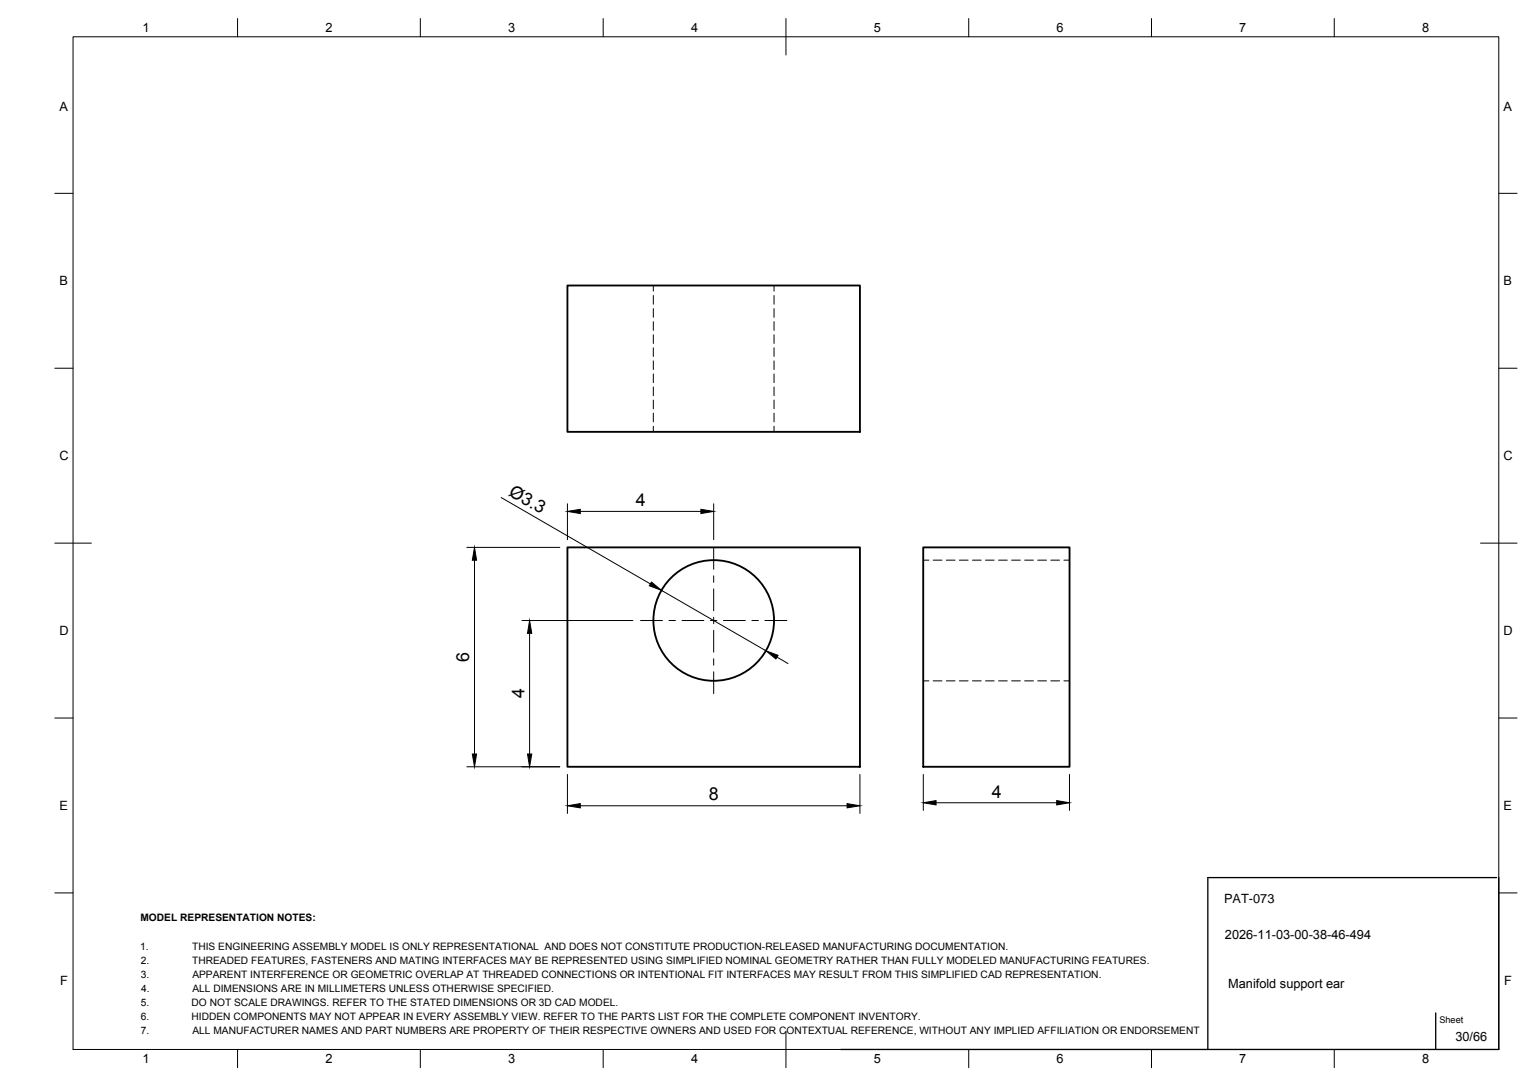
ISO-10303-21;
HEADER;
/* Generated by software containing ST-Developer
 * from STEP Tools, Inc. (www.steptools.com) 
 */

FILE_DESCRIPTION(
/* description */ ('Manual piston pump'),
/* implementation_level */ '2;1');

FILE_NAME(
/* name */ 'Manifold support ear.step',
/* time_stamp */ '2026-11-02T16:54:23-08:00',
/* author */ (''),
/* organization */ (''),
/* preprocessor_version */ 'ST-DEVELOPER v20.2',
/* originating_system */ 'Autodesk Translation Framework v15.17.0.0',
/* authorisation */ '');

FILE_SCHEMA (('AUTOMOTIVE_DESIGN { 1 0 10303 214 3 1 1 }'));
ENDSEC;

DATA;
#10=MECHANICAL_DESIGN_GEOMETRIC_PRESENTATION_REPRESENTATION('',(#732),#19043);
#598=SHAPE_REPRESENTATION_RELATIONSHIP('SRR','None',#19346,#661);
#661=ADVANCED_BREP_SHAPE_REPRESENTATION('',(#802),#19013);
#732=STYLED_ITEM('',(#19661),#802);
#802=MANIFOLD_SOLID_BREP('Body1',#9518);
#993=FACE_BOUND('',#2411,.T.);
#994=FACE_BOUND('',#2413,.T.);
#1230=CYLINDRICAL_SURFACE('',#11012,0.165);
#1664=FACE_OUTER_BOUND('',#2405,.T.);
#1665=FACE_OUTER_BOUND('',#2406,.T.);
#1666=FACE_OUTER_BOUND('',#2407,.T.);
#1667=FACE_OUTER_BOUND('',#2408,.T.);
#1668=FACE_OUTER_BOUND('',#2409,.T.);
#1669=FACE_OUTER_BOUND('',#2410,.T.);
#1670=FACE_OUTER_BOUND('',#2412,.T.);
#2405=EDGE_LOOP('',(#7799,#7800,#7801,#7802));
#2406=EDGE_LOOP('',(#7803,#7804,#7805,#7806));
#2407=EDGE_LOOP('',(#7807,#7808,#7809,#7810));
#2408=EDGE_LOOP('',(#7811,#7812,#7813,#7814));
#2409=EDGE_LOOP('',(#7815,#7816,#7817,#7818));
#2410=EDGE_LOOP('',(#7819,#7820,#7821,#7822));
#2411=EDGE_LOOP('',(#7823));
#2412=EDGE_LOOP('',(#7824,#7825,#7826,#7827));
#2413=EDGE_LOOP('',(#7828));
#3007=CIRCLE('',#11013,0.165);
#3008=CIRCLE('',#11014,0.165);
#3520=LINE('',#17795,#4124);
#3521=LINE('',#17800,#4125);
#3522=LINE('',#17802,#4126);
#3523=LINE('',#17804,#4127);
#3524=LINE('',#17805,#4128);
#3525=LINE('',#17808,#4129);
#3526=LINE('',#17810,#4130);
#3527=LINE('',#17811,#4131);
#3528=LINE('',#17814,#4132);
#3529=LINE('',#17816,#4133);
#3530=LINE('',#17817,#4134);
#3531=LINE('',#17819,#4135);
#3532=LINE('',#17820,#4136);
#4124=VECTOR('',#13410,0.165);
#4125=VECTOR('',#13415,1.);
#4126=VECTOR('',#13416,1.);
#4127=VECTOR('',#13417,1.);
#4128=VECTOR('',#13418,1.);
#4129=VECTOR('',#13421,1.);
#4130=VECTOR('',#13422,1.);
#4131=VECTOR('',#13423,1.);
#4132=VECTOR('',#13426,1.);
#4133=VECTOR('',#13427,1.);
#4134=VECTOR('',#13428,1.);
#4135=VECTOR('',#13431,1.);
#4136=VECTOR('',#13432,1.);
#4870=VERTEX_POINT('',#17792);
#4871=VERTEX_POINT('',#17794);
#4872=VERTEX_POINT('',#17798);
#4873=VERTEX_POINT('',#17799);
#4874=VERTEX_POINT('',#17801);
#4875=VERTEX_POINT('',#17803);
#4876=VERTEX_POINT('',#17807);
#4877=VERTEX_POINT('',#17809);
#4878=VERTEX_POINT('',#17813);
#4879=VERTEX_POINT('',#17815);
#5886=EDGE_CURVE('',#4870,#4870,#3007,.T.);
#5887=EDGE_CURVE('',#4870,#4871,#3520,.T.);
#5888=EDGE_CURVE('',#4871,#4871,#3008,.T.);
#5889=EDGE_CURVE('',#4872,#4873,#3521,.T.);
#5890=EDGE_CURVE('',#4873,#4874,#3522,.T.);
#5891=EDGE_CURVE('',#4875,#4874,#3523,.T.);
#5892=EDGE_CURVE('',#4872,#4875,#3524,.T.);
#5893=EDGE_CURVE('',#4876,#4872,#3525,.T.);
#5894=EDGE_CURVE('',#4877,#4875,#3526,.T.);
#5895=EDGE_CURVE('',#4876,#4877,#3527,.T.);
#5896=EDGE_CURVE('',#4878,#4876,#3528,.T.);
#5897=EDGE_CURVE('',#4879,#4877,#3529,.T.);
#5898=EDGE_CURVE('',#4878,#4879,#3530,.T.);
#5899=EDGE_CURVE('',#4873,#4878,#3531,.T.);
#5900=EDGE_CURVE('',#4874,#4879,#3532,.T.);
#7799=ORIENTED_EDGE('',*,*,#5886,.F.);
#7800=ORIENTED_EDGE('',*,*,#5887,.T.);
#7801=ORIENTED_EDGE('',*,*,#5888,.F.);
#7802=ORIENTED_EDGE('',*,*,#5887,.F.);
#7803=ORIENTED_EDGE('',*,*,#5889,.T.);
#7804=ORIENTED_EDGE('',*,*,#5890,.T.);
#7805=ORIENTED_EDGE('',*,*,#5891,.F.);
#7806=ORIENTED_EDGE('',*,*,#5892,.F.);
#7807=ORIENTED_EDGE('',*,*,#5893,.T.);
#7808=ORIENTED_EDGE('',*,*,#5892,.T.);
#7809=ORIENTED_EDGE('',*,*,#5894,.F.);
#7810=ORIENTED_EDGE('',*,*,#5895,.F.);
#7811=ORIENTED_EDGE('',*,*,#5896,.T.);
#7812=ORIENTED_EDGE('',*,*,#5895,.T.);
#7813=ORIENTED_EDGE('',*,*,#5897,.F.);
#7814=ORIENTED_EDGE('',*,*,#5898,.F.);
#7815=ORIENTED_EDGE('',*,*,#5899,.T.);
#7816=ORIENTED_EDGE('',*,*,#5898,.T.);
#7817=ORIENTED_EDGE('',*,*,#5900,.F.);
#7818=ORIENTED_EDGE('',*,*,#5890,.F.);
#7819=ORIENTED_EDGE('',*,*,#5900,.T.);
#7820=ORIENTED_EDGE('',*,*,#5897,.T.);
#7821=ORIENTED_EDGE('',*,*,#5894,.T.);
#7822=ORIENTED_EDGE('',*,*,#5891,.T.);
#7823=ORIENTED_EDGE('',*,*,#5888,.T.);
#7824=ORIENTED_EDGE('',*,*,#5899,.F.);
#7825=ORIENTED_EDGE('',*,*,#5889,.F.);
#7826=ORIENTED_EDGE('',*,*,#5893,.F.);
#7827=ORIENTED_EDGE('',*,*,#5896,.F.);
#7828=ORIENTED_EDGE('',*,*,#5886,.T.);
#8769=PLANE('',#11015);
#8770=PLANE('',#11016);
#8771=PLANE('',#11017);
#8772=PLANE('',#11018);
#8773=PLANE('',#11019);
#8774=PLANE('',#11020);
#9269=ADVANCED_FACE('',(#1664),#1230,.F.);
#9270=ADVANCED_FACE('',(#1665),#8769,.T.);
#9271=ADVANCED_FACE('',(#1666),#8770,.T.);
#9272=ADVANCED_FACE('',(#1667),#8771,.T.);
#9273=ADVANCED_FACE('',(#1668),#8772,.T.);
#9274=ADVANCED_FACE('',(#1669,#993),#8773,.T.);
#9275=ADVANCED_FACE('',(#1670,#994),#8774,.F.);
#9518=CLOSED_SHELL('',(#9269,#9270,#9271,#9272,#9273,#9274,#9275));
#11011=AXIS2_PLACEMENT_3D('',#17790,#13404,#13405);
#11012=AXIS2_PLACEMENT_3D('',#17791,#13406,#13407);
#11013=AXIS2_PLACEMENT_3D('',#17793,#13408,#13409);
#11014=AXIS2_PLACEMENT_3D('',#17796,#13411,#13412);
#11015=AXIS2_PLACEMENT_3D('',#17797,#13413,#13414);
#11016=AXIS2_PLACEMENT_3D('',#17806,#13419,#13420);
#11017=AXIS2_PLACEMENT_3D('',#17812,#13424,#13425);
#11018=AXIS2_PLACEMENT_3D('',#17818,#13429,#13430);
#11019=AXIS2_PLACEMENT_3D('',#17821,#13433,#13434);
#11020=AXIS2_PLACEMENT_3D('',#17822,#13435,#13436);
#13404=DIRECTION('axis',(0.,0.,1.));
#13405=DIRECTION('refdir',(1.,0.,0.));
#13406=DIRECTION('center_axis',(0.,0.,1.));
#13407=DIRECTION('ref_axis',(1.,0.,0.));
#13408=DIRECTION('center_axis',(0.,0.,1.));
#13409=DIRECTION('ref_axis',(1.,0.,0.));
#13410=DIRECTION('',(0.,0.,1.));
#13411=DIRECTION('center_axis',(0.,0.,-1.));
#13412=DIRECTION('ref_axis',(1.,0.,0.));
#13413=DIRECTION('center_axis',(0.,1.,0.));
#13414=DIRECTION('ref_axis',(-1.,0.,0.));
#13415=DIRECTION('',(-1.,0.,0.));
#13416=DIRECTION('',(0.,0.,1.));
#13417=DIRECTION('',(-1.,0.,0.));
#13418=DIRECTION('',(0.,0.,1.));
#13419=DIRECTION('center_axis',(1.,0.,0.));
#13420=DIRECTION('ref_axis',(0.,1.,0.));
#13421=DIRECTION('',(0.,1.,0.));
#13422=DIRECTION('',(0.,1.,0.));
#13423=DIRECTION('',(0.,0.,1.));
#13424=DIRECTION('center_axis',(0.,-1.,0.));
#13425=DIRECTION('ref_axis',(1.,0.,0.));
#13426=DIRECTION('',(1.,0.,0.));
#13427=DIRECTION('',(1.,0.,0.));
#13428=DIRECTION('',(0.,0.,1.));
#13429=DIRECTION('center_axis',(-1.,0.,0.));
#13430=DIRECTION('ref_axis',(0.,-1.,0.));
#13431=DIRECTION('',(0.,-1.,0.));
#13432=DIRECTION('',(0.,-1.,0.));
#13433=DIRECTION('center_axis',(0.,0.,1.));
#13434=DIRECTION('ref_axis',(1.,0.,0.));
#13435=DIRECTION('center_axis',(0.,0.,1.));
#13436=DIRECTION('ref_axis',(1.,0.,0.));
#17790=CARTESIAN_POINT('',(0.,0.,0.));
#17791=CARTESIAN_POINT('Origin',(-0.7,10.7,6.5));
#17792=CARTESIAN_POINT('',(-0.865,10.7,6.6));
#17793=CARTESIAN_POINT('Origin',(-0.7,10.7,6.6));
#17794=CARTESIAN_POINT('',(-0.865,10.7,7.));
#17795=CARTESIAN_POINT('',(-0.865,10.7,6.5));
#17796=CARTESIAN_POINT('Origin',(-0.7,10.7,7.));
#17797=CARTESIAN_POINT('Origin',(-0.3,10.9,6.6));
#17798=CARTESIAN_POINT('',(-0.3,10.9,6.6));
#17799=CARTESIAN_POINT('',(-1.1,10.9,6.6));
#17800=CARTESIAN_POINT('',(-0.3,10.9,6.6));
#17801=CARTESIAN_POINT('',(-1.1,10.9,7.));
#17802=CARTESIAN_POINT('',(-1.1,10.9,6.6));
#17803=CARTESIAN_POINT('',(-0.3,10.9,7.));
#17804=CARTESIAN_POINT('',(-0.3,10.9,7.));
#17805=CARTESIAN_POINT('',(-0.3,10.9,6.6));
#17806=CARTESIAN_POINT('Origin',(-0.3,10.3,6.6));
#17807=CARTESIAN_POINT('',(-0.3,10.3,6.6));
#17808=CARTESIAN_POINT('',(-0.3,10.3,6.6));
#17809=CARTESIAN_POINT('',(-0.3,10.3,7.));
#17810=CARTESIAN_POINT('',(-0.3,10.3,7.));
#17811=CARTESIAN_POINT('',(-0.3,10.3,6.6));
#17812=CARTESIAN_POINT('Origin',(-1.1,10.3,6.6));
#17813=CARTESIAN_POINT('',(-1.1,10.3,6.6));
#17814=CARTESIAN_POINT('',(-1.1,10.3,6.6));
#17815=CARTESIAN_POINT('',(-1.1,10.3,7.));
#17816=CARTESIAN_POINT('',(-1.1,10.3,7.));
#17817=CARTESIAN_POINT('',(-1.1,10.3,6.6));
#17818=CARTESIAN_POINT('Origin',(-1.1,10.9,6.6));
#17819=CARTESIAN_POINT('',(-1.1,10.9,6.6));
#17820=CARTESIAN_POINT('',(-1.1,10.9,7.));
#17821=CARTESIAN_POINT('Origin',(-0.7,10.6,7.));
#17822=CARTESIAN_POINT('Origin',(-0.7,10.6,6.6));
#18942=UNCERTAINTY_MEASURE_WITH_UNIT(LENGTH_MEASURE(0.001),#19044,
'DISTANCE_ACCURACY_VALUE',
'Maximum model space distance between geometric entities at asserted c
onnectivities');
#18972=UNCERTAINTY_MEASURE_WITH_UNIT(LENGTH_MEASURE(0.001),#19044,
'DISTANCE_ACCURACY_VALUE',
'Maximum model space distance between geometric entities at asserted c
onnectivities');
#19013=(
GEOMETRIC_REPRESENTATION_CONTEXT(3)
GLOBAL_UNCERTAINTY_ASSIGNED_CONTEXT((#18942))
GLOBAL_UNIT_ASSIGNED_CONTEXT((#19044,#19046,#19047))
REPRESENTATION_CONTEXT('','3D')
);
#19043=(
GEOMETRIC_REPRESENTATION_CONTEXT(3)
GLOBAL_UNCERTAINTY_ASSIGNED_CONTEXT((#18972))
GLOBAL_UNIT_ASSIGNED_CONTEXT((#19044,#19046,#19047))
REPRESENTATION_CONTEXT('','3D')
);
#19044=(
LENGTH_UNIT()
NAMED_UNIT(*)
SI_UNIT(.CENTI.,.METRE.)
);
#19046=(
NAMED_UNIT(*)
PLANE_ANGLE_UNIT()
SI_UNIT($,.RADIAN.)
);
#19047=(
NAMED_UNIT(*)
SI_UNIT($,.STERADIAN.)
SOLID_ANGLE_UNIT()
);
#19088=SHAPE_DEFINITION_REPRESENTATION(#19165,#19346);
#19165=PRODUCT_DEFINITION_SHAPE('',$,#19417);
#19346=SHAPE_REPRESENTATION('',(#11011),#19013);
#19376=PRODUCT_DEFINITION_CONTEXT('part definition',#19588,'design');
#19417=PRODUCT_DEFINITION('2026-11-03-00-38-46-494',
'Manifold support ear',#19487,#19376);
#19487=PRODUCT_DEFINITION_FORMATION('',$,#19630);
#19588=APPLICATION_CONTEXT(
'Core Data for Automotive Mechanical Design Process');
#19589=PRODUCT_CONTEXT('part definition',#19588,'mechanical');
#19630=PRODUCT('2026-11-03-00-38-46-494','Manifold support ear',
'Manifold support ear',(#19589));
#19661=PRESENTATION_STYLE_ASSIGNMENT((#19667));
#19667=SURFACE_STYLE_USAGE(.BOTH.,#19673);
#19673=SURFACE_SIDE_STYLE('',(#19679));
#19679=SURFACE_STYLE_FILL_AREA(#19685);
#19685=FILL_AREA_STYLE('CAD Library Painted - Engineering blue',(#19691));
#19691=FILL_AREA_STYLE_COLOUR('CAD Library Painted - Engineering blue',
#19697);
#19697=COLOUR_RGB('CAD Library Painted - Engineering blue',0.12156862745098,
0.356862745098039,0.6);
ENDSEC;
END-ISO-10303-21;
